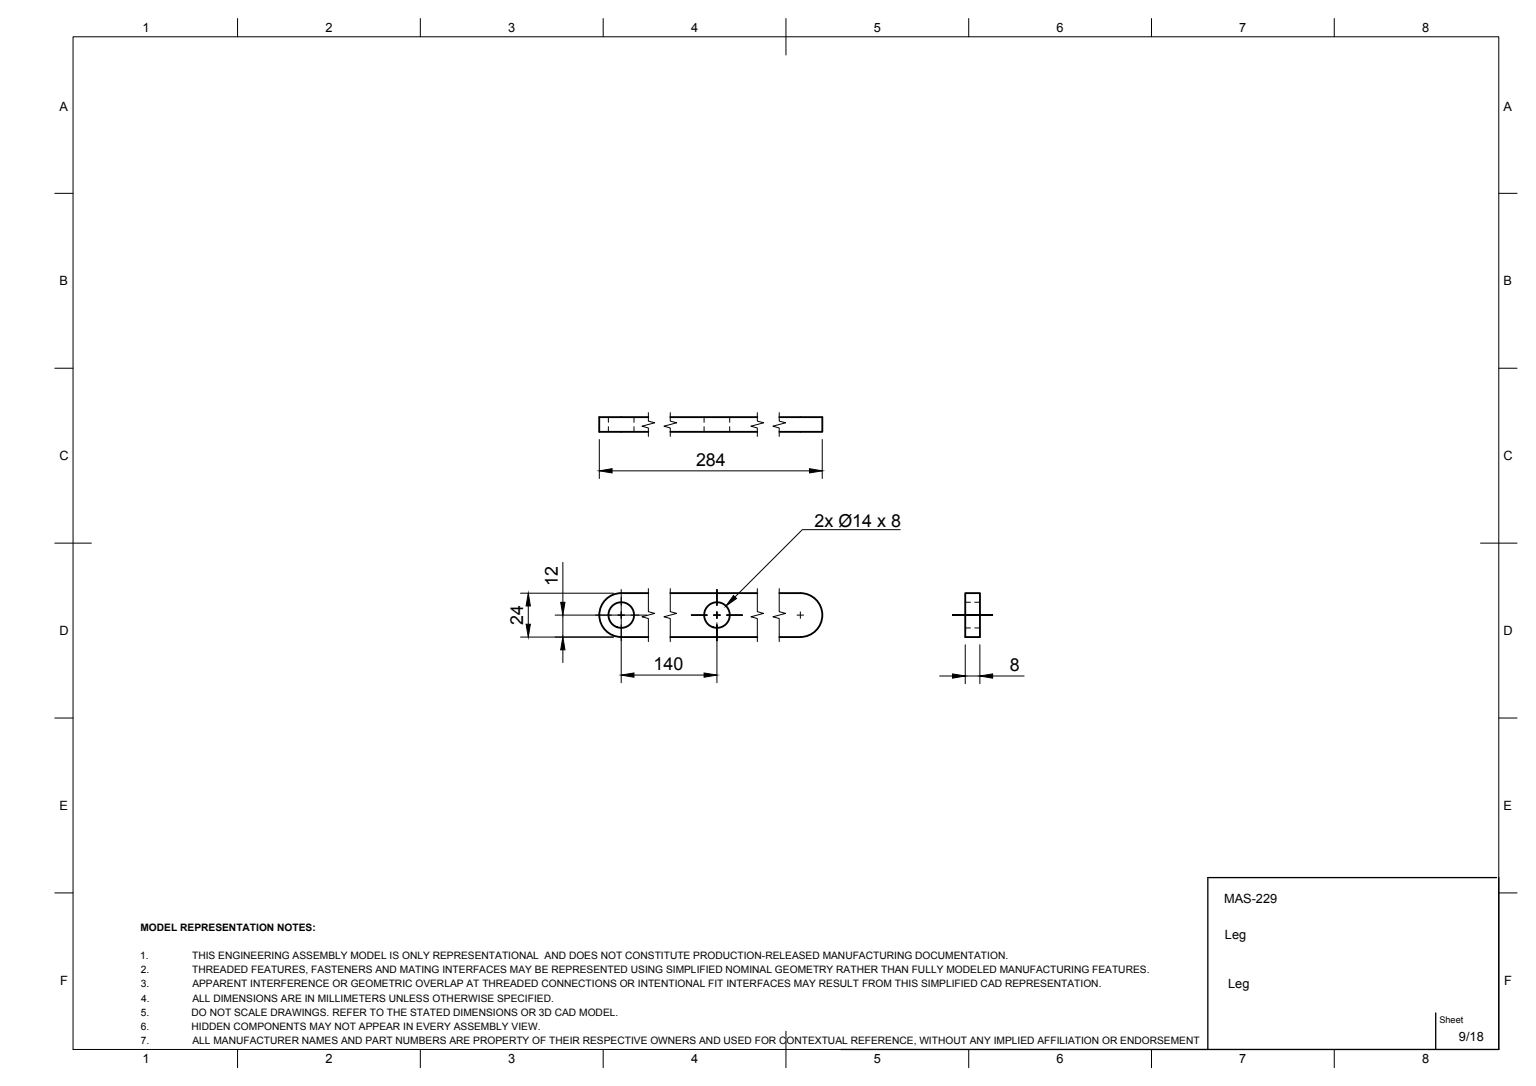
ISO-10303-21;
HEADER;
/* Generated by software containing ST-Developer
 * from STEP Tools, Inc. (www.steptools.com) 
 */

FILE_DESCRIPTION(
/* description */ ('Independently dimensioned six-bar single-leg walking-linkage demonstr
ator. Whole-mm20 crank,60 upper rocker,80/120 ternary coupler,120 lowe
r rocker,140 knee pitch and260 toe reach; ground pivots0/0,60/0,40/60.
 Seven native revolutes close both loops. Four reused native library f
amilies, fully retained shared pins and layered real spacer stacks, bo
nded rubber toe. Benchtop reference mechanism; no complete vehicle, lo
ad, gait stability, adhesive, weld, fit or life rating.'),
/* implementation_level */ '2;1');

FILE_NAME(
/* name */ 'Leg.step',
/* time_stamp */ '2026-11-09T20:33:14-08:00',
/* author */ (''),
/* organization */ (''),
/* preprocessor_version */ 'ST-DEVELOPER v20.2',
/* originating_system */ 'Autodesk Translation Framework v15.17.0.0',
/* authorisation */ '');

FILE_SCHEMA (('AUTOMOTIVE_DESIGN { 1 0 10303 214 3 1 1 }'));
ENDSEC;

DATA;
#10=MECHANICAL_DESIGN_GEOMETRIC_PRESENTATION_REPRESENTATION('',(#261),#4048);
#225=SHAPE_REPRESENTATION_RELATIONSHIP('SRR','None',#4149,#243);
#243=ADVANCED_BREP_SHAPE_REPRESENTATION('',(#279),#4036);
#261=STYLED_ITEM('',(#4248),#279);
#279=MANIFOLD_SOLID_BREP('Body1',#2150);
#323=FACE_BOUND('',#634,.T.);
#324=FACE_BOUND('',#635,.T.);
#325=FACE_BOUND('',#637,.T.);
#326=FACE_BOUND('',#638,.T.);
#378=PLANE('',#2477);
#379=PLANE('',#2481);
#380=PLANE('',#2485);
#381=PLANE('',#2486);
#469=FACE_OUTER_BOUND('',#627,.T.);
#470=FACE_OUTER_BOUND('',#628,.T.);
#471=FACE_OUTER_BOUND('',#629,.T.);
#472=FACE_OUTER_BOUND('',#630,.T.);
#473=FACE_OUTER_BOUND('',#631,.T.);
#474=FACE_OUTER_BOUND('',#632,.T.);
#475=FACE_OUTER_BOUND('',#633,.T.);
#476=FACE_OUTER_BOUND('',#636,.T.);
#627=EDGE_LOOP('',(#1737,#1738,#1739,#1740));
#628=EDGE_LOOP('',(#1741,#1742,#1743,#1744));
#629=EDGE_LOOP('',(#1745,#1746,#1747,#1748));
#630=EDGE_LOOP('',(#1749,#1750,#1751,#1752));
#631=EDGE_LOOP('',(#1753,#1754,#1755,#1756));
#632=EDGE_LOOP('',(#1757,#1758,#1759,#1760));
#633=EDGE_LOOP('',(#1761,#1762,#1763,#1764));
#634=EDGE_LOOP('',(#1765));
#635=EDGE_LOOP('',(#1766));
#636=EDGE_LOOP('',(#1767,#1768,#1769,#1770));
#637=EDGE_LOOP('',(#1771));
#638=EDGE_LOOP('',(#1772));
#802=LINE('',#3692,#927);
#803=LINE('',#3698,#928);
#804=LINE('',#3703,#929);
#805=LINE('',#3705,#930);
#806=LINE('',#3707,#931);
#807=LINE('',#3708,#932);
#808=LINE('',#3714,#933);
#809=LINE('',#3717,#934);
#810=LINE('',#3719,#935);
#811=LINE('',#3720,#936);
#927=VECTOR('',#2973,7.);
#928=VECTOR('',#2980,7.);
#929=VECTOR('',#2985,10.);
#930=VECTOR('',#2986,10.);
#931=VECTOR('',#2987,10.);
#932=VECTOR('',#2988,10.);
#933=VECTOR('',#2995,10.);
#934=VECTOR('',#2998,10.);
#935=VECTOR('',#2999,10.);
#936=VECTOR('',#3000,10.);
#1022=CIRCLE('',#2472,7.);
#1023=CIRCLE('',#2473,7.);
#1024=CIRCLE('',#2475,7.);
#1025=CIRCLE('',#2476,7.);
#1026=CIRCLE('',#2479,12.);
#1027=CIRCLE('',#2480,12.);
#1028=CIRCLE('',#2483,12.);
#1029=CIRCLE('',#2484,12.);
#1172=VERTEX_POINT('',#3689);
#1173=VERTEX_POINT('',#3691);
#1174=VERTEX_POINT('',#3695);
#1175=VERTEX_POINT('',#3697);
#1176=VERTEX_POINT('',#3701);
#1177=VERTEX_POINT('',#3702);
#1178=VERTEX_POINT('',#3704);
#1179=VERTEX_POINT('',#3706);
#1180=VERTEX_POINT('',#3710);
#1181=VERTEX_POINT('',#3712);
#1182=VERTEX_POINT('',#3716);
#1183=VERTEX_POINT('',#3718);
#1372=EDGE_CURVE('',#1172,#1172,#1022,.T.);
#1373=EDGE_CURVE('',#1172,#1173,#802,.T.);
#1374=EDGE_CURVE('',#1173,#1173,#1023,.T.);
#1375=EDGE_CURVE('',#1174,#1174,#1024,.T.);
#1376=EDGE_CURVE('',#1174,#1175,#803,.T.);
#1377=EDGE_CURVE('',#1175,#1175,#1025,.T.);
#1378=EDGE_CURVE('',#1176,#1177,#804,.T.);
#1379=EDGE_CURVE('',#1177,#1178,#805,.T.);
#1380=EDGE_CURVE('',#1179,#1178,#806,.T.);
#1381=EDGE_CURVE('',#1176,#1179,#807,.T.);
#1382=EDGE_CURVE('',#1180,#1176,#1026,.T.);
#1383=EDGE_CURVE('',#1181,#1179,#1027,.T.);
#1384=EDGE_CURVE('',#1180,#1181,#808,.T.);
#1385=EDGE_CURVE('',#1182,#1180,#809,.T.);
#1386=EDGE_CURVE('',#1183,#1181,#810,.T.);
#1387=EDGE_CURVE('',#1182,#1183,#811,.T.);
#1388=EDGE_CURVE('',#1177,#1182,#1028,.T.);
#1389=EDGE_CURVE('',#1178,#1183,#1029,.T.);
#1737=ORIENTED_EDGE('',*,*,#1372,.F.);
#1738=ORIENTED_EDGE('',*,*,#1373,.T.);
#1739=ORIENTED_EDGE('',*,*,#1374,.F.);
#1740=ORIENTED_EDGE('',*,*,#1373,.F.);
#1741=ORIENTED_EDGE('',*,*,#1375,.F.);
#1742=ORIENTED_EDGE('',*,*,#1376,.T.);
#1743=ORIENTED_EDGE('',*,*,#1377,.F.);
#1744=ORIENTED_EDGE('',*,*,#1376,.F.);
#1745=ORIENTED_EDGE('',*,*,#1378,.T.);
#1746=ORIENTED_EDGE('',*,*,#1379,.T.);
#1747=ORIENTED_EDGE('',*,*,#1380,.F.);
#1748=ORIENTED_EDGE('',*,*,#1381,.F.);
#1749=ORIENTED_EDGE('',*,*,#1382,.T.);
#1750=ORIENTED_EDGE('',*,*,#1381,.T.);
#1751=ORIENTED_EDGE('',*,*,#1383,.F.);
#1752=ORIENTED_EDGE('',*,*,#1384,.F.);
#1753=ORIENTED_EDGE('',*,*,#1385,.T.);
#1754=ORIENTED_EDGE('',*,*,#1384,.T.);
#1755=ORIENTED_EDGE('',*,*,#1386,.F.);
#1756=ORIENTED_EDGE('',*,*,#1387,.F.);
#1757=ORIENTED_EDGE('',*,*,#1388,.T.);
#1758=ORIENTED_EDGE('',*,*,#1387,.T.);
#1759=ORIENTED_EDGE('',*,*,#1389,.F.);
#1760=ORIENTED_EDGE('',*,*,#1379,.F.);
#1761=ORIENTED_EDGE('',*,*,#1389,.T.);
#1762=ORIENTED_EDGE('',*,*,#1386,.T.);
#1763=ORIENTED_EDGE('',*,*,#1383,.T.);
#1764=ORIENTED_EDGE('',*,*,#1380,.T.);
#1765=ORIENTED_EDGE('',*,*,#1372,.T.);
#1766=ORIENTED_EDGE('',*,*,#1375,.T.);
#1767=ORIENTED_EDGE('',*,*,#1388,.F.);
#1768=ORIENTED_EDGE('',*,*,#1378,.F.);
#1769=ORIENTED_EDGE('',*,*,#1382,.F.);
#1770=ORIENTED_EDGE('',*,*,#1385,.F.);
#1771=ORIENTED_EDGE('',*,*,#1374,.T.);
#1772=ORIENTED_EDGE('',*,*,#1377,.T.);
#1987=CYLINDRICAL_SURFACE('',#2471,7.);
#1988=CYLINDRICAL_SURFACE('',#2474,7.);
#1989=CYLINDRICAL_SURFACE('',#2478,12.);
#1990=CYLINDRICAL_SURFACE('',#2482,12.);
#2072=ADVANCED_FACE('',(#469),#1987,.F.);
#2073=ADVANCED_FACE('',(#470),#1988,.F.);
#2074=ADVANCED_FACE('',(#471),#378,.T.);
#2075=ADVANCED_FACE('',(#472),#1989,.T.);
#2076=ADVANCED_FACE('',(#473),#379,.T.);
#2077=ADVANCED_FACE('',(#474),#1990,.T.);
#2078=ADVANCED_FACE('',(#475,#323,#324),#380,.T.);
#2079=ADVANCED_FACE('',(#476,#325,#326),#381,.F.);
#2150=CLOSED_SHELL('',(#2072,#2073,#2074,#2075,#2076,#2077,#2078,#2079));
#2470=AXIS2_PLACEMENT_3D('',#3687,#2967,#2968);
#2471=AXIS2_PLACEMENT_3D('',#3688,#2969,#2970);
#2472=AXIS2_PLACEMENT_3D('',#3690,#2971,#2972);
#2473=AXIS2_PLACEMENT_3D('',#3693,#2974,#2975);
#2474=AXIS2_PLACEMENT_3D('',#3694,#2976,#2977);
#2475=AXIS2_PLACEMENT_3D('',#3696,#2978,#2979);
#2476=AXIS2_PLACEMENT_3D('',#3699,#2981,#2982);
#2477=AXIS2_PLACEMENT_3D('',#3700,#2983,#2984);
#2478=AXIS2_PLACEMENT_3D('',#3709,#2989,#2990);
#2479=AXIS2_PLACEMENT_3D('',#3711,#2991,#2992);
#2480=AXIS2_PLACEMENT_3D('',#3713,#2993,#2994);
#2481=AXIS2_PLACEMENT_3D('',#3715,#2996,#2997);
#2482=AXIS2_PLACEMENT_3D('',#3721,#3001,#3002);
#2483=AXIS2_PLACEMENT_3D('',#3722,#3003,#3004);
#2484=AXIS2_PLACEMENT_3D('',#3723,#3005,#3006);
#2485=AXIS2_PLACEMENT_3D('',#3724,#3007,#3008);
#2486=AXIS2_PLACEMENT_3D('',#3725,#3009,#3010);
#2967=DIRECTION('axis',(0.,0.,1.));
#2968=DIRECTION('refdir',(1.,0.,0.));
#2969=DIRECTION('center_axis',(0.,0.,-1.));
#2970=DIRECTION('ref_axis',(1.,0.,0.));
#2971=DIRECTION('center_axis',(0.,0.,-1.));
#2972=DIRECTION('ref_axis',(1.,0.,0.));
#2973=DIRECTION('',(0.,0.,-1.));
#2974=DIRECTION('center_axis',(0.,0.,1.));
#2975=DIRECTION('ref_axis',(1.,0.,0.));
#2976=DIRECTION('center_axis',(0.,0.,-1.));
#2977=DIRECTION('ref_axis',(1.,0.,0.));
#2978=DIRECTION('center_axis',(0.,0.,-1.));
#2979=DIRECTION('ref_axis',(1.,0.,0.));
#2980=DIRECTION('',(0.,0.,-1.));
#2981=DIRECTION('center_axis',(0.,0.,1.));
#2982=DIRECTION('ref_axis',(1.,0.,0.));
#2983=DIRECTION('center_axis',(0.,1.,0.));
#2984=DIRECTION('ref_axis',(-1.,0.,0.));
#2985=DIRECTION('',(-1.,0.,0.));
#2986=DIRECTION('',(0.,0.,1.));
#2987=DIRECTION('',(-1.,0.,0.));
#2988=DIRECTION('',(0.,0.,1.));
#2989=DIRECTION('center_axis',(0.,0.,1.));
#2990=DIRECTION('ref_axis',(0.,-1.,0.));
#2991=DIRECTION('center_axis',(0.,0.,1.));
#2992=DIRECTION('ref_axis',(0.,-1.,0.));
#2993=DIRECTION('center_axis',(0.,0.,1.));
#2994=DIRECTION('ref_axis',(0.,-1.,0.));
#2995=DIRECTION('',(0.,0.,1.));
#2996=DIRECTION('center_axis',(0.,-1.,0.));
#2997=DIRECTION('ref_axis',(1.,0.,0.));
#2998=DIRECTION('',(1.,0.,0.));
#2999=DIRECTION('',(1.,0.,0.));
#3000=DIRECTION('',(0.,0.,1.));
#3001=DIRECTION('center_axis',(0.,0.,1.));
#3002=DIRECTION('ref_axis',(0.,1.,0.));
#3003=DIRECTION('center_axis',(0.,0.,1.));
#3004=DIRECTION('ref_axis',(0.,1.,0.));
#3005=DIRECTION('center_axis',(0.,0.,1.));
#3006=DIRECTION('ref_axis',(0.,1.,0.));
#3007=DIRECTION('center_axis',(0.,0.,1.));
#3008=DIRECTION('ref_axis',(1.,0.,0.));
#3009=DIRECTION('center_axis',(0.,0.,1.));
#3010=DIRECTION('ref_axis',(1.,0.,0.));
#3687=CARTESIAN_POINT('',(0.,0.,0.));
#3688=CARTESIAN_POINT('Origin',(0.,0.,4.));
#3689=CARTESIAN_POINT('',(-7.,8.57252759403147E-16,8.));
#3690=CARTESIAN_POINT('Origin',(0.,0.,8.));
#3691=CARTESIAN_POINT('',(-7.,8.57252759403147E-16,0.));
#3692=CARTESIAN_POINT('',(-7.,8.57252759403147E-16,4.));
#3693=CARTESIAN_POINT('Origin',(0.,0.,0.));
#3694=CARTESIAN_POINT('Origin',(140.,0.,4.));
#3695=CARTESIAN_POINT('',(133.,8.57252759403147E-16,8.));
#3696=CARTESIAN_POINT('Origin',(140.,0.,8.));
#3697=CARTESIAN_POINT('',(133.,8.57252759403147E-16,0.));
#3698=CARTESIAN_POINT('',(133.,8.57252759403147E-16,4.));
#3699=CARTESIAN_POINT('Origin',(140.,0.,0.));
#3700=CARTESIAN_POINT('Origin',(260.,12.,0.));
#3701=CARTESIAN_POINT('',(260.,12.,0.));
#3702=CARTESIAN_POINT('',(0.,12.,0.));
#3703=CARTESIAN_POINT('',(260.,12.,0.));
#3704=CARTESIAN_POINT('',(0.,12.,8.));
#3705=CARTESIAN_POINT('',(0.,12.,0.));
#3706=CARTESIAN_POINT('',(260.,12.,8.));
#3707=CARTESIAN_POINT('',(260.,12.,8.));
#3708=CARTESIAN_POINT('',(260.,12.,0.));
#3709=CARTESIAN_POINT('Origin',(260.,-1.11022302462516E-15,0.));
#3710=CARTESIAN_POINT('',(260.,-12.,0.));
#3711=CARTESIAN_POINT('Origin',(260.,-1.11022302462516E-15,0.));
#3712=CARTESIAN_POINT('',(260.,-12.,8.));
#3713=CARTESIAN_POINT('Origin',(260.,-1.11022302462516E-15,8.));
#3714=CARTESIAN_POINT('',(260.,-12.,0.));
#3715=CARTESIAN_POINT('Origin',(0.,-12.,0.));
#3716=CARTESIAN_POINT('',(-1.46957615897682E-15,-12.,0.));
#3717=CARTESIAN_POINT('',(0.,-12.,0.));
#3718=CARTESIAN_POINT('',(-1.46957615897682E-15,-12.,8.));
#3719=CARTESIAN_POINT('',(0.,-12.,8.));
#3720=CARTESIAN_POINT('',(-1.46957615897682E-15,-12.,0.));
#3721=CARTESIAN_POINT('Origin',(0.,0.,0.));
#3722=CARTESIAN_POINT('Origin',(0.,0.,0.));
#3723=CARTESIAN_POINT('Origin',(0.,0.,8.));
#3724=CARTESIAN_POINT('Origin',(130.,0.,8.));
#3725=CARTESIAN_POINT('Origin',(130.,0.,0.));
#4016=UNCERTAINTY_MEASURE_WITH_UNIT(LENGTH_MEASURE(0.01),#4049,
'DISTANCE_ACCURACY_VALUE',
'Maximum model space distance between geometric entities at asserted c
onnectivities');
#4028=UNCERTAINTY_MEASURE_WITH_UNIT(LENGTH_MEASURE(0.01),#4049,
'DISTANCE_ACCURACY_VALUE',
'Maximum model space distance between geometric entities at asserted c
onnectivities');
#4036=(
GEOMETRIC_REPRESENTATION_CONTEXT(3)
GLOBAL_UNCERTAINTY_ASSIGNED_CONTEXT((#4016))
GLOBAL_UNIT_ASSIGNED_CONTEXT((#4049,#4051,#4052))
REPRESENTATION_CONTEXT('','3D')
);
#4048=(
GEOMETRIC_REPRESENTATION_CONTEXT(3)
GLOBAL_UNCERTAINTY_ASSIGNED_CONTEXT((#4028))
GLOBAL_UNIT_ASSIGNED_CONTEXT((#4049,#4051,#4052))
REPRESENTATION_CONTEXT('','3D')
);
#4049=(
LENGTH_UNIT()
NAMED_UNIT(*)
SI_UNIT(.MILLI.,.METRE.)
);
#4051=(
NAMED_UNIT(*)
PLANE_ANGLE_UNIT()
SI_UNIT($,.RADIAN.)
);
#4052=(
NAMED_UNIT(*)
SI_UNIT($,.STERADIAN.)
SOLID_ANGLE_UNIT()
);
#4060=SHAPE_DEFINITION_REPRESENTATION(#4079,#4149);
#4079=PRODUCT_DEFINITION_SHAPE('',$,#4169);
#4149=SHAPE_REPRESENTATION('',(#2470),#4036);
#4161=PRODUCT_DEFINITION_CONTEXT('part definition',#4220,'design');
#4169=PRODUCT_DEFINITION('Leg','Leg',#4188,#4161);
#4188=PRODUCT_DEFINITION_FORMATION('',$,#4229);
#4220=APPLICATION_CONTEXT(
'Core Data for Automotive Mechanical Design Process');
#4221=PRODUCT_CONTEXT('part definition',#4220,'mechanical');
#4229=PRODUCT('Leg','Leg',$,(#4221));
#4248=PRESENTATION_STYLE_ASSIGNMENT((#4262));
#4262=SURFACE_STYLE_USAGE(.BOTH.,#4276);
#4276=SURFACE_SIDE_STYLE('',(#4290));
#4290=SURFACE_STYLE_FILL_AREA(#4304);
#4304=FILL_AREA_STYLE('Leg finish',(#4318));
#4318=FILL_AREA_STYLE_COLOUR('Leg finish',#4332);
#4332=COLOUR_RGB('Leg finish',0.0901960784313725,0.270588235294118,0.513725490196078);
ENDSEC;
END-ISO-10303-21;
